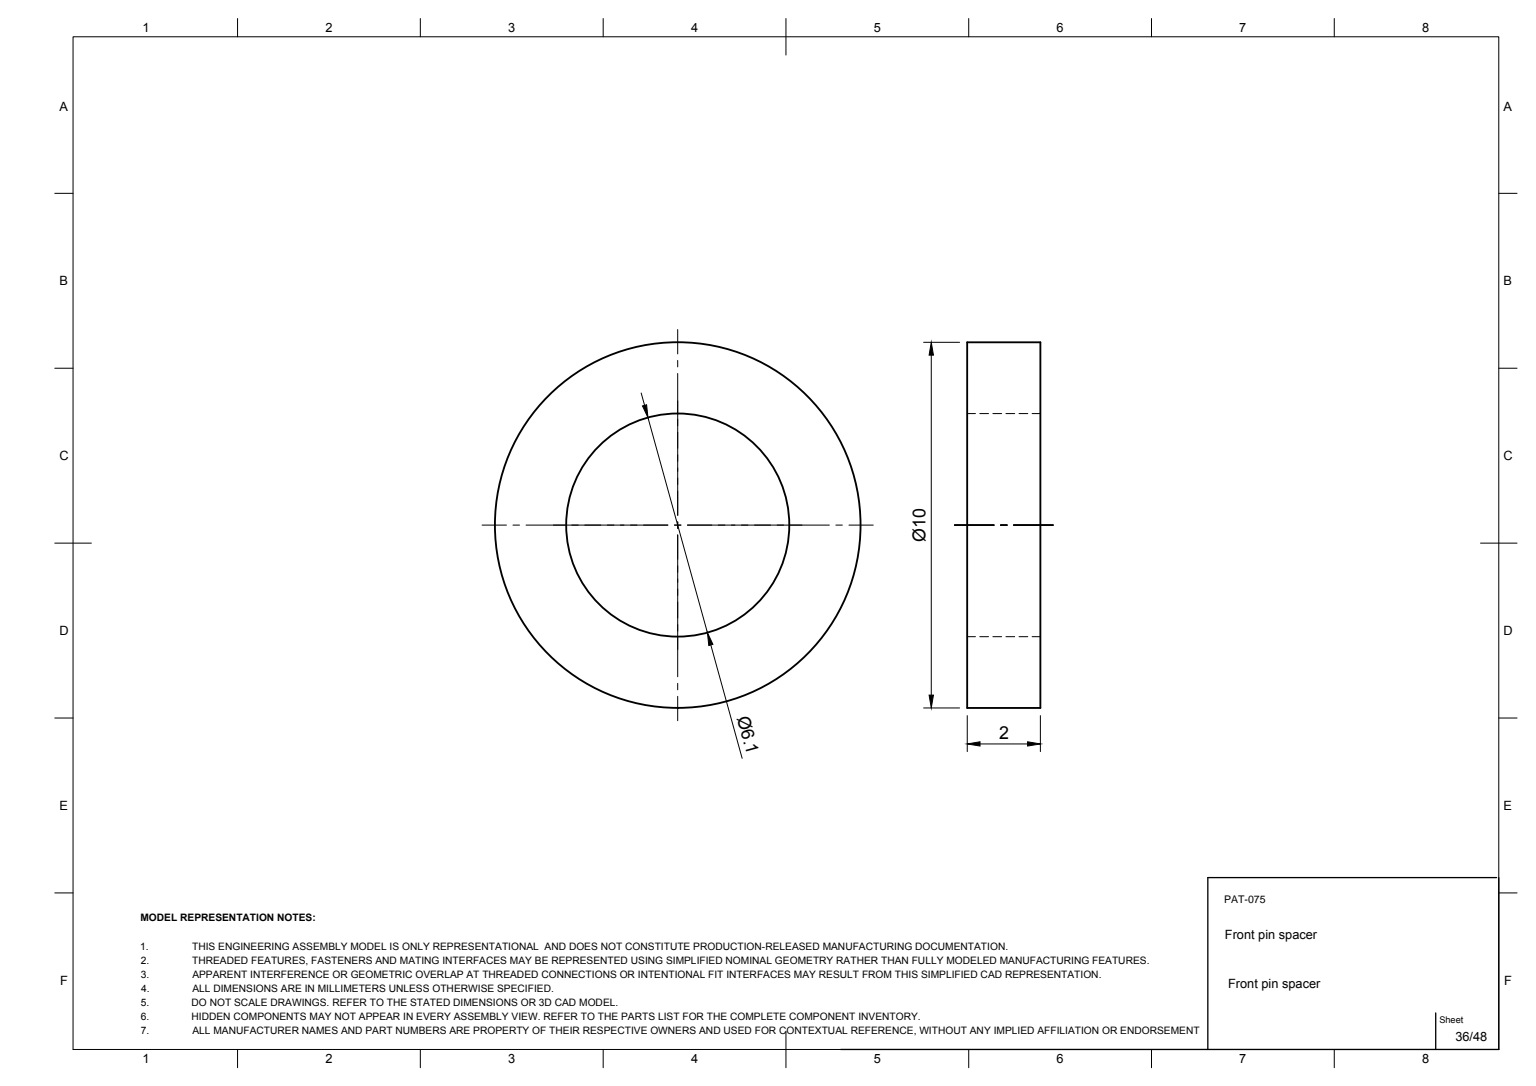
ISO-10303-21;
HEADER;
/* Generated by software containing ST-Developer
 * from STEP Tools, Inc. (www.steptools.com) 
 */

FILE_DESCRIPTION(
/* description */ ('Over-Centre Plunger Toggle Clamp on Slotted Fixture Frame'),
/* implementation_level */ '2;1');

FILE_NAME(
/* name */ 
'Front pin spacer.step',
/* time_stamp */ '2026-10-28T03:23:24-07:00',
/* author */ (''),
/* organization */ (''),
/* preprocessor_version */ 'ST-DEVELOPER v20.2',
/* originating_system */ 'Autodesk Translation Framework v15.17.0.0',
/* authorisation */ '');

FILE_SCHEMA (('AUTOMOTIVE_DESIGN { 1 0 10303 214 3 1 1 }'));
ENDSEC;

DATA;
#10=MECHANICAL_DESIGN_GEOMETRIC_PRESENTATION_REPRESENTATION('',(#550),#15212);
#458=SHAPE_REPRESENTATION_RELATIONSHIP('SRR','None',#15435,#500);
#500=ADVANCED_BREP_SHAPE_REPRESENTATION('',(#599),#15197);
#550=STYLED_ITEM('',(#15719),#599);
#599=MANIFOLD_SOLID_BREP('Body1',#8284);
#759=FACE_BOUND('',#2094,.T.);
#760=FACE_BOUND('',#2096,.T.);
#1009=PLANE('',#9480);
#1010=PLANE('',#9481);
#1457=FACE_OUTER_BOUND('',#2091,.T.);
#1458=FACE_OUTER_BOUND('',#2092,.T.);
#1459=FACE_OUTER_BOUND('',#2093,.T.);
#1460=FACE_OUTER_BOUND('',#2095,.T.);
#2091=EDGE_LOOP('',(#7171,#7172,#7173,#7174));
#2092=EDGE_LOOP('',(#7175,#7176,#7177,#7178));
#2093=EDGE_LOOP('',(#7179));
#2094=EDGE_LOOP('',(#7180));
#2095=EDGE_LOOP('',(#7181));
#2096=EDGE_LOOP('',(#7182));
#2711=LINE('',#14522,#3341);
#2712=LINE('',#14528,#3342);
#3341=VECTOR('',#11660,0.305);
#3342=VECTOR('',#11667,0.5);
#3788=CIRCLE('',#9475,0.305);
#3789=CIRCLE('',#9476,0.305);
#3790=CIRCLE('',#9478,0.5);
#3791=CIRCLE('',#9479,0.5);
#4400=VERTEX_POINT('',#14519);
#4401=VERTEX_POINT('',#14521);
#4402=VERTEX_POINT('',#14525);
#4403=VERTEX_POINT('',#14527);
#5346=EDGE_CURVE('',#4400,#4400,#3788,.T.);
#5347=EDGE_CURVE('',#4400,#4401,#2711,.T.);
#5348=EDGE_CURVE('',#4401,#4401,#3789,.T.);
#5349=EDGE_CURVE('',#4402,#4402,#3790,.T.);
#5350=EDGE_CURVE('',#4402,#4403,#2712,.T.);
#5351=EDGE_CURVE('',#4403,#4403,#3791,.T.);
#7171=ORIENTED_EDGE('',*,*,#5346,.F.);
#7172=ORIENTED_EDGE('',*,*,#5347,.T.);
#7173=ORIENTED_EDGE('',*,*,#5348,.T.);
#7174=ORIENTED_EDGE('',*,*,#5347,.F.);
#7175=ORIENTED_EDGE('',*,*,#5349,.F.);
#7176=ORIENTED_EDGE('',*,*,#5350,.T.);
#7177=ORIENTED_EDGE('',*,*,#5351,.T.);
#7178=ORIENTED_EDGE('',*,*,#5350,.F.);
#7179=ORIENTED_EDGE('',*,*,#5349,.T.);
#7180=ORIENTED_EDGE('',*,*,#5346,.T.);
#7181=ORIENTED_EDGE('',*,*,#5351,.F.);
#7182=ORIENTED_EDGE('',*,*,#5348,.F.);
#7731=CYLINDRICAL_SURFACE('',#9474,0.305);
#7732=CYLINDRICAL_SURFACE('',#9477,0.5);
#8129=ADVANCED_FACE('',(#1457),#7731,.F.);
#8130=ADVANCED_FACE('',(#1458),#7732,.T.);
#8131=ADVANCED_FACE('',(#1459,#759),#1009,.T.);
#8132=ADVANCED_FACE('',(#1460,#760),#1010,.F.);
#8284=CLOSED_SHELL('',(#8129,#8130,#8131,#8132));
#9473=AXIS2_PLACEMENT_3D('',#14517,#11654,#11655);
#9474=AXIS2_PLACEMENT_3D('',#14518,#11656,#11657);
#9475=AXIS2_PLACEMENT_3D('',#14520,#11658,#11659);
#9476=AXIS2_PLACEMENT_3D('',#14523,#11661,#11662);
#9477=AXIS2_PLACEMENT_3D('',#14524,#11663,#11664);
#9478=AXIS2_PLACEMENT_3D('',#14526,#11665,#11666);
#9479=AXIS2_PLACEMENT_3D('',#14529,#11668,#11669);
#9480=AXIS2_PLACEMENT_3D('',#14530,#11670,#11671);
#9481=AXIS2_PLACEMENT_3D('',#14531,#11672,#11673);
#11654=DIRECTION('axis',(0.,0.,1.));
#11655=DIRECTION('refdir',(1.,0.,0.));
#11656=DIRECTION('center_axis',(0.,1.,0.));
#11657=DIRECTION('ref_axis',(1.,0.,0.));
#11658=DIRECTION('center_axis',(0.,-1.,0.));
#11659=DIRECTION('ref_axis',(1.,0.,0.));
#11660=DIRECTION('',(0.,-1.,0.));
#11661=DIRECTION('center_axis',(0.,-1.,0.));
#11662=DIRECTION('ref_axis',(1.,0.,0.));
#11663=DIRECTION('center_axis',(0.,1.,0.));
#11664=DIRECTION('ref_axis',(1.,0.,0.));
#11665=DIRECTION('center_axis',(0.,1.,0.));
#11666=DIRECTION('ref_axis',(1.,0.,0.));
#11667=DIRECTION('',(0.,-1.,0.));
#11668=DIRECTION('center_axis',(0.,1.,0.));
#11669=DIRECTION('ref_axis',(1.,0.,0.));
#11670=DIRECTION('center_axis',(0.,1.,0.));
#11671=DIRECTION('ref_axis',(1.,0.,0.));
#11672=DIRECTION('center_axis',(0.,1.,0.));
#11673=DIRECTION('ref_axis',(1.,0.,0.));
#14517=CARTESIAN_POINT('',(0.,0.,0.));
#14518=CARTESIAN_POINT('Origin',(-2.82632109303527,-5.7,8.79263101785268));
#14519=CARTESIAN_POINT('',(-3.13132109303527,-5.5,8.79263101785268));
#14520=CARTESIAN_POINT('Origin',(-2.82632109303527,-5.5,8.79263101785268));
#14521=CARTESIAN_POINT('',(-3.13132109303527,-5.7,8.79263101785268));
#14522=CARTESIAN_POINT('',(-3.13132109303527,-5.7,8.79263101785268));
#14523=CARTESIAN_POINT('Origin',(-2.82632109303527,-5.7,8.79263101785268));
#14524=CARTESIAN_POINT('Origin',(-2.82632109303527,-5.7,8.79263101785268));
#14525=CARTESIAN_POINT('',(-3.32632109303527,-5.5,8.79263101785268));
#14526=CARTESIAN_POINT('Origin',(-2.82632109303527,-5.5,8.79263101785268));
#14527=CARTESIAN_POINT('',(-3.32632109303527,-5.7,8.79263101785268));
#14528=CARTESIAN_POINT('',(-3.32632109303527,-5.7,8.79263101785268));
#14529=CARTESIAN_POINT('Origin',(-2.82632109303527,-5.7,8.79263101785268));
#14530=CARTESIAN_POINT('Origin',(-2.82632109303527,-5.5,8.79263101785268));
#14531=CARTESIAN_POINT('Origin',(-2.82632109303527,-5.7,8.79263101785268));
#15147=UNCERTAINTY_MEASURE_WITH_UNIT(LENGTH_MEASURE(0.001),#15213,
'DISTANCE_ACCURACY_VALUE',
'Maximum model space distance between geometric entities at asserted c
onnectivities');
#15162=UNCERTAINTY_MEASURE_WITH_UNIT(LENGTH_MEASURE(0.001),#15213,
'DISTANCE_ACCURACY_VALUE',
'Maximum model space distance between geometric entities at asserted c
onnectivities');
#15197=(
GEOMETRIC_REPRESENTATION_CONTEXT(3)
GLOBAL_UNCERTAINTY_ASSIGNED_CONTEXT((#15147))
GLOBAL_UNIT_ASSIGNED_CONTEXT((#15213,#15215,#15216))
REPRESENTATION_CONTEXT('','3D')
);
#15212=(
GEOMETRIC_REPRESENTATION_CONTEXT(3)
GLOBAL_UNCERTAINTY_ASSIGNED_CONTEXT((#15162))
GLOBAL_UNIT_ASSIGNED_CONTEXT((#15213,#15215,#15216))
REPRESENTATION_CONTEXT('','3D')
);
#15213=(
LENGTH_UNIT()
NAMED_UNIT(*)
SI_UNIT(.CENTI.,.METRE.)
);
#15215=(
NAMED_UNIT(*)
PLANE_ANGLE_UNIT()
SI_UNIT($,.RADIAN.)
);
#15216=(
NAMED_UNIT(*)
SI_UNIT($,.STERADIAN.)
SOLID_ANGLE_UNIT()
);
#15251=SHAPE_DEFINITION_REPRESENTATION(#15307,#15435);
#15307=PRODUCT_DEFINITION_SHAPE('',$,#15485);
#15435=SHAPE_REPRESENTATION('',(#9473),#15197);
#15450=PRODUCT_DEFINITION_CONTEXT('part definition',#15599,'design');
#15485=PRODUCT_DEFINITION('Front pin spacer','Front pin spacer',#15534,
#15450);
#15534=PRODUCT_DEFINITION_FORMATION('',$,#15635);
#15599=APPLICATION_CONTEXT(
'Core Data for Automotive Mechanical Design Process');
#15600=PRODUCT_CONTEXT('part definition',#15599,'mechanical');
#15635=PRODUCT('Front pin spacer','Front pin spacer','Front pin spacer',
(#15600));
#15713=COLOUR_RGB('Grey',0.48,0.52,0.57);
#15714=FILL_AREA_STYLE_COLOUR('',#15713);
#15715=FILL_AREA_STYLE('',(#15714));
#15716=SURFACE_STYLE_FILL_AREA(#15715);
#15717=SURFACE_SIDE_STYLE('',(#15716));
#15718=SURFACE_STYLE_USAGE(.BOTH.,#15717);
#15719=PRESENTATION_STYLE_ASSIGNMENT((#15718));
ENDSEC;
END-ISO-10303-21;
